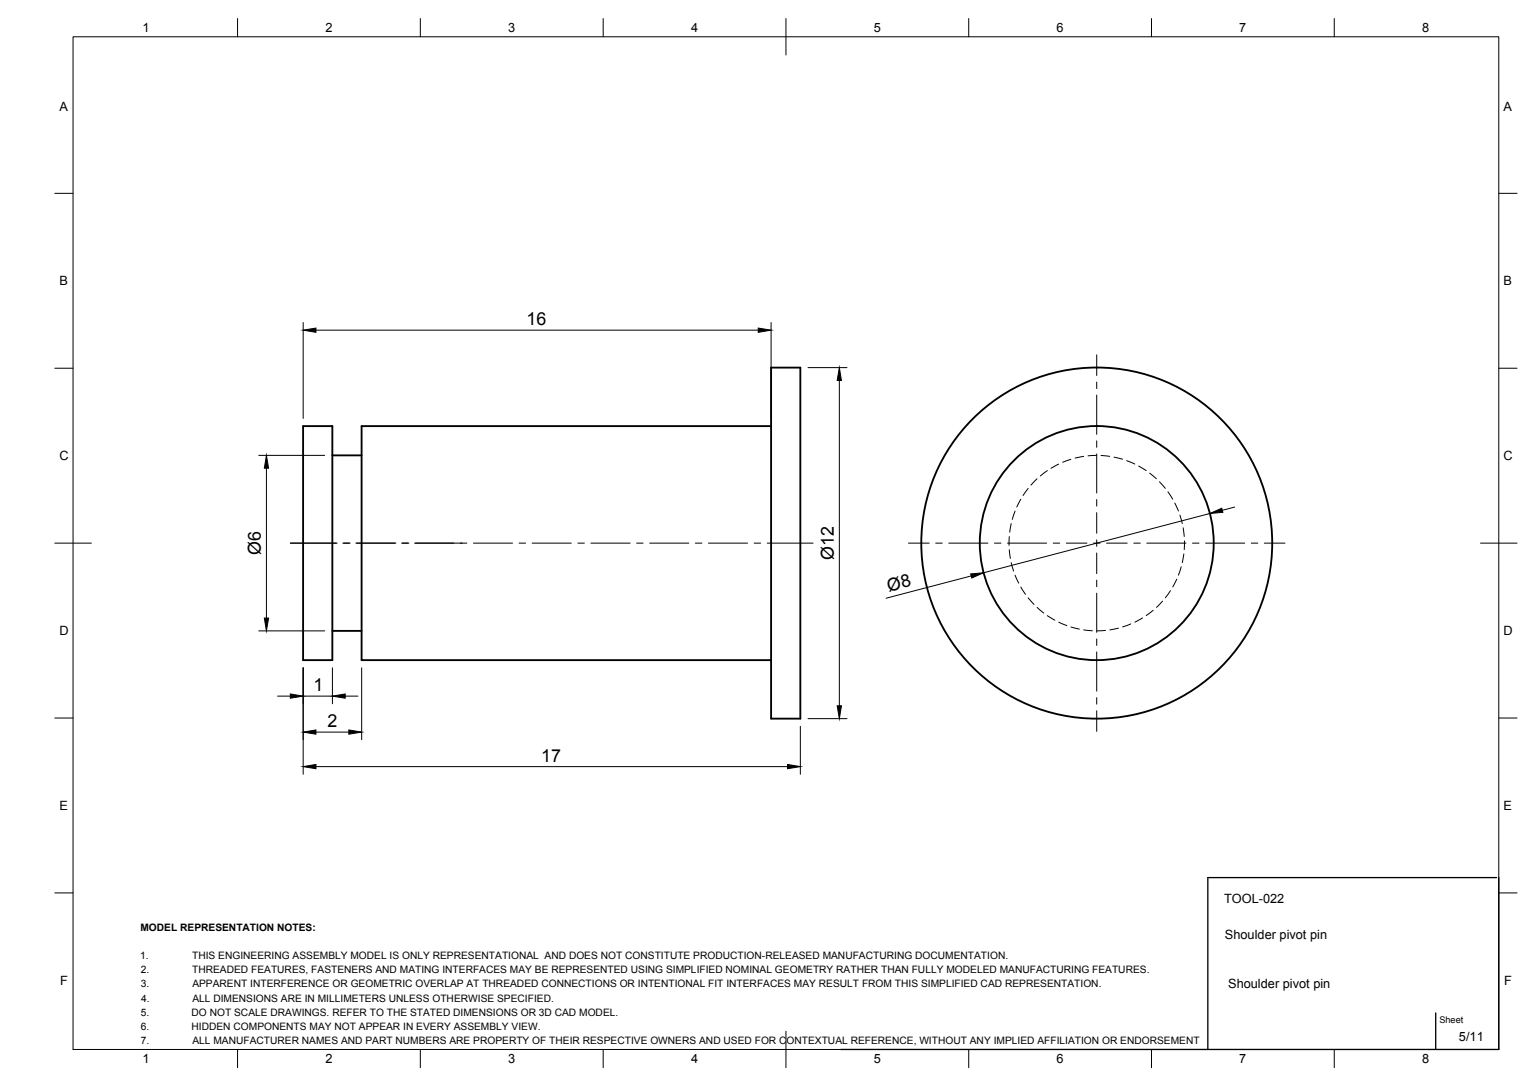
ISO-10303-21;
HEADER;
/* Generated by software containing ST-Developer
 * from STEP Tools, Inc. (www.steptools.com) 
 */

FILE_DESCRIPTION(
/* description */ (''),
/* implementation_level */ '2;1');

FILE_NAME(
/* name */ 'Shoulder pivot pin.step',
/* time_stamp */ '2026-11-10T08:27:36-08:00',
/* author */ (''),
/* organization */ (''),
/* preprocessor_version */ 'ST-DEVELOPER v20.2',
/* originating_system */ 'Autodesk Translation Framework v15.17.0.0',
/* authorisation */ '');

FILE_SCHEMA (('AUTOMOTIVE_DESIGN { 1 0 10303 214 3 1 1 }'));
ENDSEC;

DATA;
#10=MECHANICAL_DESIGN_GEOMETRIC_PRESENTATION_REPRESENTATION('',(#568),#19090);
#548=SHAPE_REPRESENTATION_RELATIONSHIP('SRR','None',#19138,#558);
#558=ADVANCED_BREP_SHAPE_REPRESENTATION('',(#578),#19081);
#568=STYLED_ITEM('',(#19201),#578);
#578=MANIFOLD_SOLID_BREP('Body1',#6822);
#598=FACE_BOUND('',#1262,.T.);
#599=FACE_BOUND('',#1264,.T.);
#600=FACE_BOUND('',#1267,.T.);
#690=PLANE('',#7015);
#691=PLANE('',#7017);
#692=PLANE('',#7021);
#693=PLANE('',#7026);
#694=PLANE('',#7028);
#860=FACE_OUTER_BOUND('',#1260,.T.);
#861=FACE_OUTER_BOUND('',#1261,.T.);
#862=FACE_OUTER_BOUND('',#1263,.T.);
#863=FACE_OUTER_BOUND('',#1265,.T.);
#864=FACE_OUTER_BOUND('',#1266,.T.);
#865=FACE_OUTER_BOUND('',#1268,.T.);
#866=FACE_OUTER_BOUND('',#1269,.T.);
#867=FACE_OUTER_BOUND('',#1270,.T.);
#868=FACE_OUTER_BOUND('',#1271,.T.);
#1260=EDGE_LOOP('',(#4585,#4586,#4587,#4588));
#1261=EDGE_LOOP('',(#4589));
#1262=EDGE_LOOP('',(#4590));
#1263=EDGE_LOOP('',(#4591));
#1264=EDGE_LOOP('',(#4592));
#1265=EDGE_LOOP('',(#4593,#4594,#4595,#4596));
#1266=EDGE_LOOP('',(#4597));
#1267=EDGE_LOOP('',(#4598));
#1268=EDGE_LOOP('',(#4599,#4600,#4601,#4602));
#1269=EDGE_LOOP('',(#4603));
#1270=EDGE_LOOP('',(#4604,#4605,#4606,#4607));
#1271=EDGE_LOOP('',(#4608));
#1761=LINE('',#9140,#2210);
#1762=LINE('',#9151,#2211);
#1763=LINE('',#9159,#2212);
#1764=LINE('',#9163,#2213);
#2210=VECTOR('',#7688,0.3);
#2211=VECTOR('',#7703,0.4);
#2212=VECTOR('',#7712,0.6);
#2213=VECTOR('',#7719,0.4);
#2574=CIRCLE('',#7013,0.3);
#2575=CIRCLE('',#7014,0.3);
#2576=CIRCLE('',#7016,0.4);
#2577=CIRCLE('',#7018,0.4);
#2578=CIRCLE('',#7020,0.4);
#2579=CIRCLE('',#7022,0.6);
#2580=CIRCLE('',#7023,0.4);
#2581=CIRCLE('',#7025,0.6);
#2796=VERTEX_POINT('',#9137);
#2797=VERTEX_POINT('',#9139);
#2798=VERTEX_POINT('',#9143);
#2799=VERTEX_POINT('',#9146);
#2800=VERTEX_POINT('',#9149);
#2801=VERTEX_POINT('',#9153);
#2802=VERTEX_POINT('',#9155);
#2803=VERTEX_POINT('',#9158);
#3477=EDGE_CURVE('',#2796,#2796,#2574,.T.);
#3478=EDGE_CURVE('',#2796,#2797,#1761,.T.);
#3479=EDGE_CURVE('',#2797,#2797,#2575,.T.);
#3480=EDGE_CURVE('',#2798,#2798,#2576,.T.);
#3481=EDGE_CURVE('',#2799,#2799,#2577,.T.);
#3482=EDGE_CURVE('',#2800,#2800,#2578,.T.);
#3483=EDGE_CURVE('',#2800,#2799,#1762,.T.);
#3484=EDGE_CURVE('',#2801,#2801,#2579,.T.);
#3485=EDGE_CURVE('',#2802,#2802,#2580,.T.);
#3486=EDGE_CURVE('',#2801,#2803,#1763,.T.);
#3487=EDGE_CURVE('',#2803,#2803,#2581,.T.);
#3488=EDGE_CURVE('',#2798,#2802,#1764,.T.);
#4585=ORIENTED_EDGE('',*,*,#3477,.T.);
#4586=ORIENTED_EDGE('',*,*,#3478,.T.);
#4587=ORIENTED_EDGE('',*,*,#3479,.F.);
#4588=ORIENTED_EDGE('',*,*,#3478,.F.);
#4589=ORIENTED_EDGE('',*,*,#3480,.F.);
#4590=ORIENTED_EDGE('',*,*,#3477,.F.);
#4591=ORIENTED_EDGE('',*,*,#3481,.F.);
#4592=ORIENTED_EDGE('',*,*,#3479,.T.);
#4593=ORIENTED_EDGE('',*,*,#3482,.F.);
#4594=ORIENTED_EDGE('',*,*,#3483,.T.);
#4595=ORIENTED_EDGE('',*,*,#3481,.T.);
#4596=ORIENTED_EDGE('',*,*,#3483,.F.);
#4597=ORIENTED_EDGE('',*,*,#3484,.T.);
#4598=ORIENTED_EDGE('',*,*,#3485,.F.);
#4599=ORIENTED_EDGE('',*,*,#3484,.F.);
#4600=ORIENTED_EDGE('',*,*,#3486,.T.);
#4601=ORIENTED_EDGE('',*,*,#3487,.T.);
#4602=ORIENTED_EDGE('',*,*,#3486,.F.);
#4603=ORIENTED_EDGE('',*,*,#3487,.F.);
#4604=ORIENTED_EDGE('',*,*,#3480,.T.);
#4605=ORIENTED_EDGE('',*,*,#3488,.T.);
#4606=ORIENTED_EDGE('',*,*,#3485,.T.);
#4607=ORIENTED_EDGE('',*,*,#3488,.F.);
#4608=ORIENTED_EDGE('',*,*,#3482,.T.);
#6311=CYLINDRICAL_SURFACE('',#7012,0.3);
#6312=CYLINDRICAL_SURFACE('',#7019,0.4);
#6313=CYLINDRICAL_SURFACE('',#7024,0.6);
#6314=CYLINDRICAL_SURFACE('',#7027,0.4);
#6479=ADVANCED_FACE('',(#860),#6311,.T.);
#6480=ADVANCED_FACE('',(#861,#598),#690,.F.);
#6481=ADVANCED_FACE('',(#862,#599),#691,.F.);
#6482=ADVANCED_FACE('',(#863),#6312,.T.);
#6483=ADVANCED_FACE('',(#864,#600),#692,.T.);
#6484=ADVANCED_FACE('',(#865),#6313,.T.);
#6485=ADVANCED_FACE('',(#866),#693,.F.);
#6486=ADVANCED_FACE('',(#867),#6314,.T.);
#6487=ADVANCED_FACE('',(#868),#694,.T.);
#6822=CLOSED_SHELL('',(#6479,#6480,#6481,#6482,#6483,#6484,#6485,#6486,
#6487));
#7011=AXIS2_PLACEMENT_3D('',#9135,#7682,#7683);
#7012=AXIS2_PLACEMENT_3D('',#9136,#7684,#7685);
#7013=AXIS2_PLACEMENT_3D('',#9138,#7686,#7687);
#7014=AXIS2_PLACEMENT_3D('',#9141,#7689,#7690);
#7015=AXIS2_PLACEMENT_3D('',#9142,#7691,#7692);
#7016=AXIS2_PLACEMENT_3D('',#9144,#7693,#7694);
#7017=AXIS2_PLACEMENT_3D('',#9145,#7695,#7696);
#7018=AXIS2_PLACEMENT_3D('',#9147,#7697,#7698);
#7019=AXIS2_PLACEMENT_3D('',#9148,#7699,#7700);
#7020=AXIS2_PLACEMENT_3D('',#9150,#7701,#7702);
#7021=AXIS2_PLACEMENT_3D('',#9152,#7704,#7705);
#7022=AXIS2_PLACEMENT_3D('',#9154,#7706,#7707);
#7023=AXIS2_PLACEMENT_3D('',#9156,#7708,#7709);
#7024=AXIS2_PLACEMENT_3D('',#9157,#7710,#7711);
#7025=AXIS2_PLACEMENT_3D('',#9160,#7713,#7714);
#7026=AXIS2_PLACEMENT_3D('',#9161,#7715,#7716);
#7027=AXIS2_PLACEMENT_3D('',#9162,#7717,#7718);
#7028=AXIS2_PLACEMENT_3D('',#9164,#7720,#7721);
#7682=DIRECTION('axis',(0.,0.,1.));
#7683=DIRECTION('refdir',(1.,0.,0.));
#7684=DIRECTION('center_axis',(0.,0.,1.));
#7685=DIRECTION('ref_axis',(1.,0.,0.));
#7686=DIRECTION('center_axis',(0.,0.,1.));
#7687=DIRECTION('ref_axis',(1.,0.,0.));
#7688=DIRECTION('',(0.,0.,1.));
#7689=DIRECTION('center_axis',(0.,0.,1.));
#7690=DIRECTION('ref_axis',(1.,0.,0.));
#7691=DIRECTION('center_axis',(0.,0.,-1.));
#7692=DIRECTION('ref_axis',(-1.,0.,0.));
#7693=DIRECTION('center_axis',(0.,0.,-1.));
#7694=DIRECTION('ref_axis',(1.,0.,0.));
#7695=DIRECTION('center_axis',(0.,0.,1.));
#7696=DIRECTION('ref_axis',(1.,0.,0.));
#7697=DIRECTION('center_axis',(0.,0.,1.));
#7698=DIRECTION('ref_axis',(1.,0.,0.));
#7699=DIRECTION('center_axis',(0.,0.,1.));
#7700=DIRECTION('ref_axis',(1.,0.,0.));
#7701=DIRECTION('center_axis',(0.,0.,1.));
#7702=DIRECTION('ref_axis',(1.,0.,0.));
#7703=DIRECTION('',(0.,0.,-1.));
#7704=DIRECTION('center_axis',(0.,0.,1.));
#7705=DIRECTION('ref_axis',(1.,0.,0.));
#7706=DIRECTION('center_axis',(0.,0.,1.));
#7707=DIRECTION('ref_axis',(1.,0.,0.));
#7708=DIRECTION('center_axis',(0.,0.,1.));
#7709=DIRECTION('ref_axis',(1.,0.,0.));
#7710=DIRECTION('center_axis',(0.,0.,1.));
#7711=DIRECTION('ref_axis',(1.,0.,0.));
#7712=DIRECTION('',(0.,0.,-1.));
#7713=DIRECTION('center_axis',(0.,0.,1.));
#7714=DIRECTION('ref_axis',(1.,0.,0.));
#7715=DIRECTION('center_axis',(0.,0.,1.));
#7716=DIRECTION('ref_axis',(1.,0.,0.));
#7717=DIRECTION('center_axis',(0.,0.,1.));
#7718=DIRECTION('ref_axis',(1.,0.,0.));
#7719=DIRECTION('',(0.,0.,-1.));
#7720=DIRECTION('center_axis',(0.,0.,1.));
#7721=DIRECTION('ref_axis',(1.,0.,0.));
#9135=CARTESIAN_POINT('',(0.,0.,0.));
#9136=CARTESIAN_POINT('Origin',(0.,0.,0.75));
#9137=CARTESIAN_POINT('',(-0.3,-3.67394039744206E-17,0.7));
#9138=CARTESIAN_POINT('Origin',(0.,0.,0.7));
#9139=CARTESIAN_POINT('',(-0.3,-3.67394039744206E-17,0.8));
#9140=CARTESIAN_POINT('',(-0.3,-3.67394039744206E-17,0.75));
#9141=CARTESIAN_POINT('Origin',(0.,0.,0.8));
#9142=CARTESIAN_POINT('Origin',(0.7,0.,0.7));
#9143=CARTESIAN_POINT('',(-0.4,4.89858719658941E-17,0.7));
#9144=CARTESIAN_POINT('Origin',(0.,0.,0.7));
#9145=CARTESIAN_POINT('Origin',(0.3,0.,0.8));
#9146=CARTESIAN_POINT('',(-0.4,-4.89858719658941E-17,0.8));
#9147=CARTESIAN_POINT('Origin',(0.,0.,0.8));
#9148=CARTESIAN_POINT('Origin',(0.,0.,-0.7));
#9149=CARTESIAN_POINT('',(-0.4,-4.89858719658941E-17,0.9));
#9150=CARTESIAN_POINT('Origin',(0.,0.,0.9));
#9151=CARTESIAN_POINT('',(-0.4,-4.89858719658941E-17,-0.7));
#9152=CARTESIAN_POINT('Origin',(0.,0.,-0.7));
#9153=CARTESIAN_POINT('',(-0.6,-7.34788079488412E-17,-0.7));
#9154=CARTESIAN_POINT('Origin',(0.,0.,-0.7));
#9155=CARTESIAN_POINT('',(-0.4,-4.89858719658941E-17,-0.7));
#9156=CARTESIAN_POINT('Origin',(0.,0.,-0.7));
#9157=CARTESIAN_POINT('Origin',(0.,0.,-0.8));
#9158=CARTESIAN_POINT('',(-0.6,-7.34788079488412E-17,-0.8));
#9159=CARTESIAN_POINT('',(-0.6,-7.34788079488412E-17,-0.8));
#9160=CARTESIAN_POINT('Origin',(0.,0.,-0.8));
#9161=CARTESIAN_POINT('Origin',(0.,0.,-0.8));
#9162=CARTESIAN_POINT('Origin',(0.,0.,-0.7));
#9163=CARTESIAN_POINT('',(-0.4,-4.89858719658941E-17,-0.7));
#9164=CARTESIAN_POINT('Origin',(0.,0.,0.9));
#19068=UNCERTAINTY_MEASURE_WITH_UNIT(LENGTH_MEASURE(0.001),#19091,
'DISTANCE_ACCURACY_VALUE',
'Maximum model space distance between geometric entities at asserted c
onnectivities');
#19077=UNCERTAINTY_MEASURE_WITH_UNIT(LENGTH_MEASURE(0.001),#19091,
'DISTANCE_ACCURACY_VALUE',
'Maximum model space distance between geometric entities at asserted c
onnectivities');
#19081=(
GEOMETRIC_REPRESENTATION_CONTEXT(3)
GLOBAL_UNCERTAINTY_ASSIGNED_CONTEXT((#19068))
GLOBAL_UNIT_ASSIGNED_CONTEXT((#19091,#19093,#19094))
REPRESENTATION_CONTEXT('','3D')
);
#19090=(
GEOMETRIC_REPRESENTATION_CONTEXT(3)
GLOBAL_UNCERTAINTY_ASSIGNED_CONTEXT((#19077))
GLOBAL_UNIT_ASSIGNED_CONTEXT((#19091,#19093,#19094))
REPRESENTATION_CONTEXT('','3D')
);
#19091=(
LENGTH_UNIT()
NAMED_UNIT(*)
SI_UNIT(.CENTI.,.METRE.)
);
#19093=(
NAMED_UNIT(*)
PLANE_ANGLE_UNIT()
SI_UNIT($,.RADIAN.)
);
#19094=(
NAMED_UNIT(*)
SI_UNIT($,.STERADIAN.)
SOLID_ANGLE_UNIT()
);
#19098=SHAPE_DEFINITION_REPRESENTATION(#19110,#19138);
#19110=PRODUCT_DEFINITION_SHAPE('',$,#19151);
#19138=SHAPE_REPRESENTATION('',(#7011),#19081);
#19147=PRODUCT_DEFINITION_CONTEXT('part definition',#19185,'design');
#19151=PRODUCT_DEFINITION('Shoulder pivot pin','Shoulder pivot pin',#19163,
#19147);
#19163=PRODUCT_DEFINITION_FORMATION('',$,#19190);
#19185=APPLICATION_CONTEXT(
'Core Data for Automotive Mechanical Design Process');
#19186=PRODUCT_CONTEXT('part definition',#19185,'mechanical');
#19190=PRODUCT('Shoulder pivot pin','Shoulder pivot pin',$,(#19186));
#19201=PRESENTATION_STYLE_ASSIGNMENT((#19209));
#19209=SURFACE_STYLE_USAGE(.BOTH.,#19217);
#19217=SURFACE_SIDE_STYLE('',(#19225));
#19225=SURFACE_STYLE_FILL_AREA(#19233);
#19233=FILL_AREA_STYLE('Pivot dark gray',(#19241));
#19241=FILL_AREA_STYLE_COLOUR('Pivot dark gray',#19249);
#19249=COLOUR_RGB('Pivot dark gray',0.27843137254902,0.309803921568627,
0.352941176470588);
ENDSEC;
END-ISO-10303-21;
